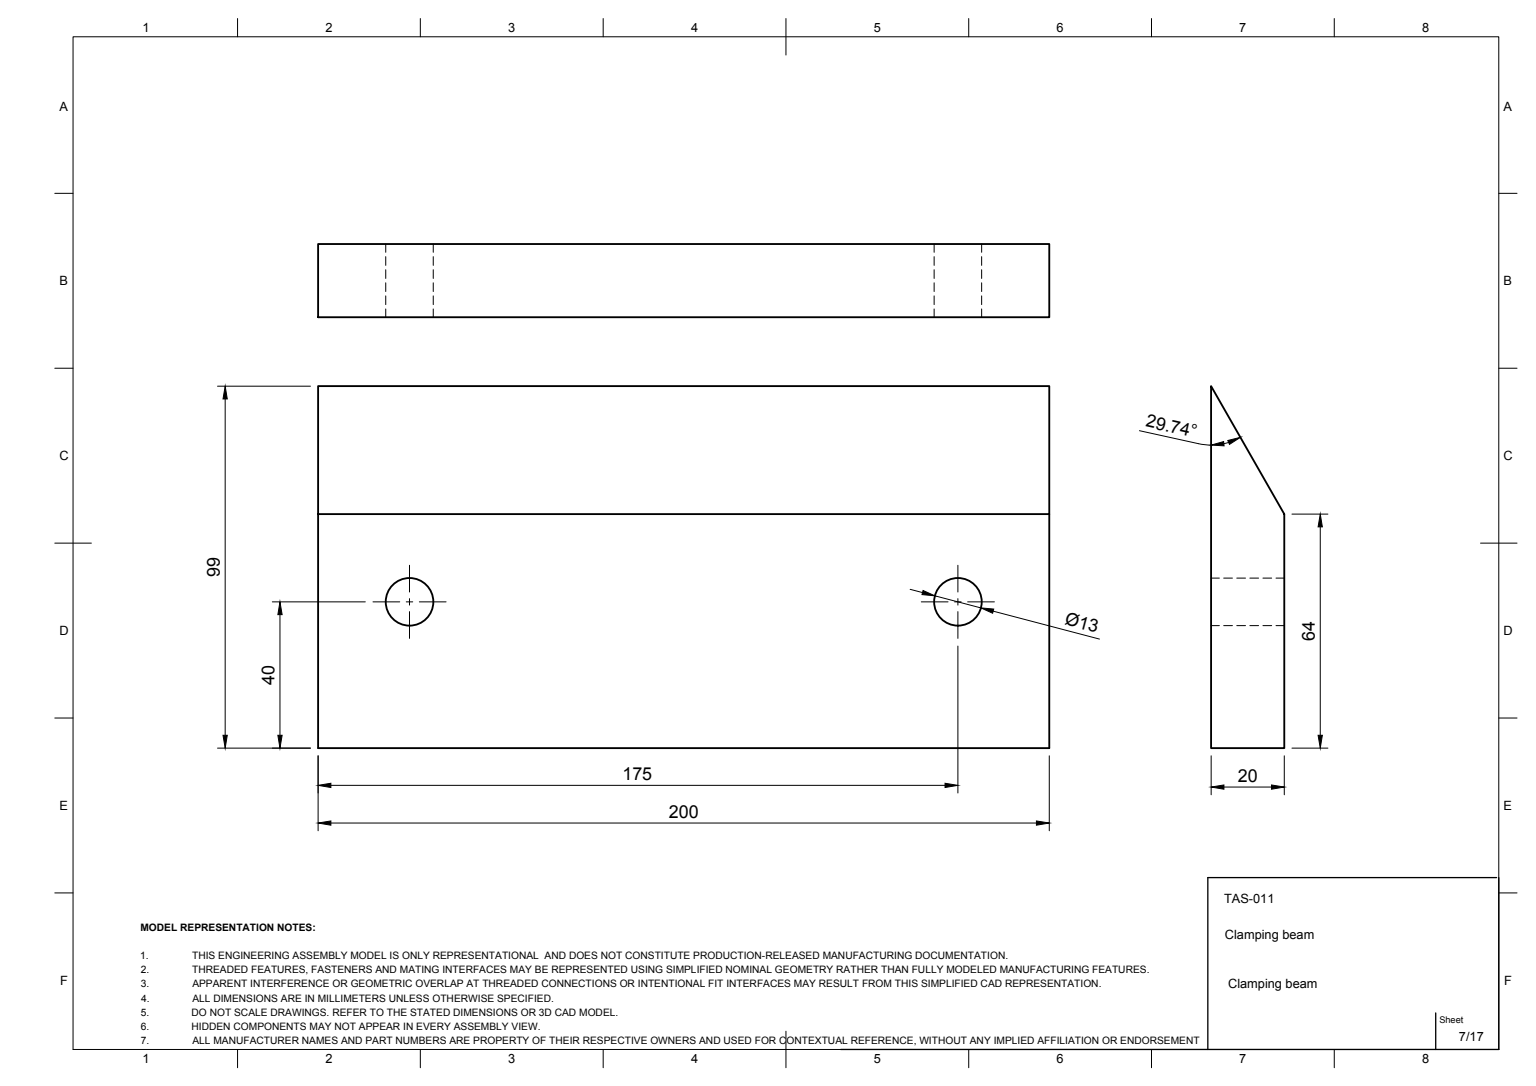
ISO-10303-21;
HEADER;
/* Generated by software containing ST-Developer
 * from STEP Tools, Inc. (www.steptools.com) 
 */

FILE_DESCRIPTION(
/* description */ (
'Independent manual bench leaf bending machine,200mm work width. Fabri
cated welded frame and folding leaf, repeated bushed and fully retaine
d hinge hardware, two handles with bonded grips, beveled clamping beam
 and modeledM12 clamp screws.2mm omitted-workpiece assembly reference 
gap, not a capacity claim. Native135deg hinge travel. Weld sizing, pro
duction fits, material condition, bending capacity, strength and life 
unassigned.'),
/* implementation_level */ '2;1');

FILE_NAME(
/* name */ 'Clamping beam.step',
/* time_stamp */ '2026-11-14T09:11:34-08:00',
/* author */ (''),
/* organization */ (''),
/* preprocessor_version */ 'ST-DEVELOPER v20.2',
/* originating_system */ 'Autodesk Translation Framework v15.17.0.0',
/* authorisation */ '');

FILE_SCHEMA (('AUTOMOTIVE_DESIGN { 1 0 10303 214 3 1 1 }'));
ENDSEC;

DATA;
#10=MECHANICAL_DESIGN_GEOMETRIC_PRESENTATION_REPRESENTATION('',(#448),#37701);
#412=SHAPE_REPRESENTATION_RELATIONSHIP('SRR','None',#37781,#430);
#430=ADVANCED_BREP_SHAPE_REPRESENTATION('',(#466),#37685);
#448=STYLED_ITEM('',(#37880),#466);
#466=MANIFOLD_SOLID_BREP('Body1',#4146);
#494=FACE_BOUND('',#852,.T.);
#495=FACE_BOUND('',#853,.T.);
#496=FACE_BOUND('',#856,.T.);
#497=FACE_BOUND('',#857,.T.);
#528=PLANE('',#4413);
#529=PLANE('',#4414);
#530=PLANE('',#4415);
#531=PLANE('',#4416);
#532=PLANE('',#4417);
#533=PLANE('',#4418);
#624=FACE_OUTER_BOUND('',#848,.T.);
#625=FACE_OUTER_BOUND('',#849,.T.);
#626=FACE_OUTER_BOUND('',#850,.T.);
#627=FACE_OUTER_BOUND('',#851,.T.);
#628=FACE_OUTER_BOUND('',#854,.T.);
#629=FACE_OUTER_BOUND('',#855,.T.);
#630=FACE_OUTER_BOUND('',#858,.T.);
#631=FACE_OUTER_BOUND('',#859,.T.);
#848=EDGE_LOOP('',(#2747,#2748,#2749,#2750));
#849=EDGE_LOOP('',(#2751,#2752,#2753,#2754));
#850=EDGE_LOOP('',(#2755,#2756,#2757,#2758));
#851=EDGE_LOOP('',(#2759,#2760,#2761,#2762));
#852=EDGE_LOOP('',(#2763));
#853=EDGE_LOOP('',(#2764));
#854=EDGE_LOOP('',(#2765,#2766,#2767,#2768));
#855=EDGE_LOOP('',(#2769,#2770,#2771,#2772));
#856=EDGE_LOOP('',(#2773));
#857=EDGE_LOOP('',(#2774));
#858=EDGE_LOOP('',(#2775,#2776,#2777,#2778));
#859=EDGE_LOOP('',(#2779,#2780,#2781,#2782));
#1094=LINE('',#5768,#1343);
#1095=LINE('',#5774,#1344);
#1096=LINE('',#5779,#1345);
#1097=LINE('',#5781,#1346);
#1098=LINE('',#5783,#1347);
#1099=LINE('',#5784,#1348);
#1100=LINE('',#5787,#1349);
#1101=LINE('',#5789,#1350);
#1102=LINE('',#5790,#1351);
#1103=LINE('',#5793,#1352);
#1104=LINE('',#5795,#1353);
#1105=LINE('',#5796,#1354);
#1106=LINE('',#5798,#1355);
#1107=LINE('',#5799,#1356);
#1343=VECTOR('',#4837,6.5);
#1344=VECTOR('',#4844,6.5);
#1345=VECTOR('',#4849,10.);
#1346=VECTOR('',#4850,10.);
#1347=VECTOR('',#4851,10.);
#1348=VECTOR('',#4852,10.);
#1349=VECTOR('',#4855,10.);
#1350=VECTOR('',#4856,10.);
#1351=VECTOR('',#4857,10.);
#1352=VECTOR('',#4860,10.);
#1353=VECTOR('',#4861,10.);
#1354=VECTOR('',#4862,10.);
#1355=VECTOR('',#4865,10.);
#1356=VECTOR('',#4866,10.);
#1578=CIRCLE('',#4408,6.5);
#1579=CIRCLE('',#4409,6.5);
#1580=CIRCLE('',#4411,6.5);
#1581=CIRCLE('',#4412,6.5);
#1673=VERTEX_POINT('',#5765);
#1674=VERTEX_POINT('',#5767);
#1675=VERTEX_POINT('',#5771);
#1676=VERTEX_POINT('',#5773);
#1677=VERTEX_POINT('',#5777);
#1678=VERTEX_POINT('',#5778);
#1679=VERTEX_POINT('',#5780);
#1680=VERTEX_POINT('',#5782);
#1681=VERTEX_POINT('',#5786);
#1682=VERTEX_POINT('',#5788);
#1683=VERTEX_POINT('',#5792);
#1684=VERTEX_POINT('',#5794);
#2107=EDGE_CURVE('',#1673,#1673,#1578,.T.);
#2108=EDGE_CURVE('',#1673,#1674,#1094,.T.);
#2109=EDGE_CURVE('',#1674,#1674,#1579,.T.);
#2110=EDGE_CURVE('',#1675,#1675,#1580,.T.);
#2111=EDGE_CURVE('',#1675,#1676,#1095,.T.);
#2112=EDGE_CURVE('',#1676,#1676,#1581,.T.);
#2113=EDGE_CURVE('',#1677,#1678,#1096,.T.);
#2114=EDGE_CURVE('',#1677,#1679,#1097,.T.);
#2115=EDGE_CURVE('',#1680,#1679,#1098,.T.);
#2116=EDGE_CURVE('',#1678,#1680,#1099,.T.);
#2117=EDGE_CURVE('',#1678,#1681,#1100,.T.);
#2118=EDGE_CURVE('',#1682,#1680,#1101,.T.);
#2119=EDGE_CURVE('',#1681,#1682,#1102,.T.);
#2120=EDGE_CURVE('',#1681,#1683,#1103,.T.);
#2121=EDGE_CURVE('',#1684,#1682,#1104,.T.);
#2122=EDGE_CURVE('',#1683,#1684,#1105,.T.);
#2123=EDGE_CURVE('',#1683,#1677,#1106,.T.);
#2124=EDGE_CURVE('',#1679,#1684,#1107,.T.);
#2747=ORIENTED_EDGE('',*,*,#2107,.F.);
#2748=ORIENTED_EDGE('',*,*,#2108,.T.);
#2749=ORIENTED_EDGE('',*,*,#2109,.F.);
#2750=ORIENTED_EDGE('',*,*,#2108,.F.);
#2751=ORIENTED_EDGE('',*,*,#2110,.F.);
#2752=ORIENTED_EDGE('',*,*,#2111,.T.);
#2753=ORIENTED_EDGE('',*,*,#2112,.F.);
#2754=ORIENTED_EDGE('',*,*,#2111,.F.);
#2755=ORIENTED_EDGE('',*,*,#2113,.F.);
#2756=ORIENTED_EDGE('',*,*,#2114,.T.);
#2757=ORIENTED_EDGE('',*,*,#2115,.F.);
#2758=ORIENTED_EDGE('',*,*,#2116,.F.);
#2759=ORIENTED_EDGE('',*,*,#2117,.F.);
#2760=ORIENTED_EDGE('',*,*,#2116,.T.);
#2761=ORIENTED_EDGE('',*,*,#2118,.F.);
#2762=ORIENTED_EDGE('',*,*,#2119,.F.);
#2763=ORIENTED_EDGE('',*,*,#2109,.T.);
#2764=ORIENTED_EDGE('',*,*,#2112,.T.);
#2765=ORIENTED_EDGE('',*,*,#2120,.F.);
#2766=ORIENTED_EDGE('',*,*,#2119,.T.);
#2767=ORIENTED_EDGE('',*,*,#2121,.F.);
#2768=ORIENTED_EDGE('',*,*,#2122,.F.);
#2769=ORIENTED_EDGE('',*,*,#2123,.F.);
#2770=ORIENTED_EDGE('',*,*,#2122,.T.);
#2771=ORIENTED_EDGE('',*,*,#2124,.F.);
#2772=ORIENTED_EDGE('',*,*,#2114,.F.);
#2773=ORIENTED_EDGE('',*,*,#2107,.T.);
#2774=ORIENTED_EDGE('',*,*,#2110,.T.);
#2775=ORIENTED_EDGE('',*,*,#2124,.T.);
#2776=ORIENTED_EDGE('',*,*,#2121,.T.);
#2777=ORIENTED_EDGE('',*,*,#2118,.T.);
#2778=ORIENTED_EDGE('',*,*,#2115,.T.);
#2779=ORIENTED_EDGE('',*,*,#2123,.T.);
#2780=ORIENTED_EDGE('',*,*,#2113,.T.);
#2781=ORIENTED_EDGE('',*,*,#2117,.T.);
#2782=ORIENTED_EDGE('',*,*,#2120,.T.);
#3821=CYLINDRICAL_SURFACE('',#4407,6.5);
#3822=CYLINDRICAL_SURFACE('',#4410,6.5);
#3954=ADVANCED_FACE('',(#624),#3821,.F.);
#3955=ADVANCED_FACE('',(#625),#3822,.F.);
#3956=ADVANCED_FACE('',(#626),#528,.T.);
#3957=ADVANCED_FACE('',(#627,#494,#495),#529,.T.);
#3958=ADVANCED_FACE('',(#628),#530,.T.);
#3959=ADVANCED_FACE('',(#629,#496,#497),#531,.T.);
#3960=ADVANCED_FACE('',(#630),#532,.T.);
#3961=ADVANCED_FACE('',(#631),#533,.F.);
#4146=CLOSED_SHELL('',(#3954,#3955,#3956,#3957,#3958,#3959,#3960,#3961));
#4406=AXIS2_PLACEMENT_3D('',#5763,#4831,#4832);
#4407=AXIS2_PLACEMENT_3D('',#5764,#4833,#4834);
#4408=AXIS2_PLACEMENT_3D('',#5766,#4835,#4836);
#4409=AXIS2_PLACEMENT_3D('',#5769,#4838,#4839);
#4410=AXIS2_PLACEMENT_3D('',#5770,#4840,#4841);
#4411=AXIS2_PLACEMENT_3D('',#5772,#4842,#4843);
#4412=AXIS2_PLACEMENT_3D('',#5775,#4845,#4846);
#4413=AXIS2_PLACEMENT_3D('',#5776,#4847,#4848);
#4414=AXIS2_PLACEMENT_3D('',#5785,#4853,#4854);
#4415=AXIS2_PLACEMENT_3D('',#5791,#4858,#4859);
#4416=AXIS2_PLACEMENT_3D('',#5797,#4863,#4864);
#4417=AXIS2_PLACEMENT_3D('',#5800,#4867,#4868);
#4418=AXIS2_PLACEMENT_3D('',#5801,#4869,#4870);
#4831=DIRECTION('axis',(0.,0.,1.));
#4832=DIRECTION('refdir',(1.,0.,0.));
#4833=DIRECTION('center_axis',(0.,0.,-1.));
#4834=DIRECTION('ref_axis',(1.,0.,0.));
#4835=DIRECTION('center_axis',(0.,0.,-1.));
#4836=DIRECTION('ref_axis',(1.,0.,0.));
#4837=DIRECTION('',(0.,0.,-1.));
#4838=DIRECTION('center_axis',(0.,0.,1.));
#4839=DIRECTION('ref_axis',(1.,0.,0.));
#4840=DIRECTION('center_axis',(0.,0.,-1.));
#4841=DIRECTION('ref_axis',(1.,0.,0.));
#4842=DIRECTION('center_axis',(0.,0.,-1.));
#4843=DIRECTION('ref_axis',(1.,0.,0.));
#4844=DIRECTION('',(0.,0.,-1.));
#4845=DIRECTION('center_axis',(0.,0.,1.));
#4846=DIRECTION('ref_axis',(1.,0.,0.));
#4847=DIRECTION('center_axis',(-1.,0.,0.));
#4848=DIRECTION('ref_axis',(0.,0.,1.));
#4849=DIRECTION('',(0.,0.,-1.));
#4850=DIRECTION('',(0.,1.,0.));
#4851=DIRECTION('',(0.,0.,1.));
#4852=DIRECTION('',(0.,1.,0.));
#4853=DIRECTION('center_axis',(0.,0.,-1.));
#4854=DIRECTION('ref_axis',(-1.,0.,0.));
#4855=DIRECTION('',(1.,0.,0.));
#4856=DIRECTION('',(-1.,0.,0.));
#4857=DIRECTION('',(0.,1.,0.));
#4858=DIRECTION('center_axis',(0.496138938356834,0.,0.868243142124459));
#4859=DIRECTION('ref_axis',(0.868243142124459,0.,-0.496138938356834));
#4860=DIRECTION('',(-0.868243142124459,0.,0.496138938356834));
#4861=DIRECTION('',(0.868243142124459,0.,-0.496138938356834));
#4862=DIRECTION('',(0.,1.,0.));
#4863=DIRECTION('center_axis',(0.,0.,1.));
#4864=DIRECTION('ref_axis',(1.,0.,0.));
#4865=DIRECTION('',(-1.,0.,0.));
#4866=DIRECTION('',(1.,0.,0.));
#4867=DIRECTION('center_axis',(0.,1.,0.));
#4868=DIRECTION('ref_axis',(0.,0.,1.));
#4869=DIRECTION('center_axis',(0.,1.,0.));
#4870=DIRECTION('ref_axis',(1.,0.,0.));
#5763=CARTESIAN_POINT('',(0.,0.,0.));
#5764=CARTESIAN_POINT('Origin',(-60.,25.,52.));
#5765=CARTESIAN_POINT('',(-66.5,25.,62.));
#5766=CARTESIAN_POINT('Origin',(-60.,25.,62.));
#5767=CARTESIAN_POINT('',(-66.5,25.,42.));
#5768=CARTESIAN_POINT('',(-66.5,25.,52.));
#5769=CARTESIAN_POINT('Origin',(-60.,25.,42.));
#5770=CARTESIAN_POINT('Origin',(-60.,175.,52.));
#5771=CARTESIAN_POINT('',(-66.5,175.,62.));
#5772=CARTESIAN_POINT('Origin',(-60.,175.,62.));
#5773=CARTESIAN_POINT('',(-66.5,175.,42.));
#5774=CARTESIAN_POINT('',(-66.5,175.,52.));
#5775=CARTESIAN_POINT('Origin',(-60.,175.,42.));
#5776=CARTESIAN_POINT('Origin',(-100.,0.,42.));
#5777=CARTESIAN_POINT('',(-100.,0.,62.));
#5778=CARTESIAN_POINT('',(-100.,0.,42.));
#5779=CARTESIAN_POINT('',(-100.,0.,62.));
#5780=CARTESIAN_POINT('',(-100.,200.,62.));
#5781=CARTESIAN_POINT('',(-100.,0.,62.));
#5782=CARTESIAN_POINT('',(-100.,200.,42.));
#5783=CARTESIAN_POINT('',(-100.,200.,62.));
#5784=CARTESIAN_POINT('',(-100.,0.,42.));
#5785=CARTESIAN_POINT('Origin',(-0.999999999999996,0.,42.));
#5786=CARTESIAN_POINT('',(-1.,0.,42.));
#5787=CARTESIAN_POINT('',(-100.,0.,42.));
#5788=CARTESIAN_POINT('',(-1.,200.,42.));
#5789=CARTESIAN_POINT('',(-100.,200.,42.));
#5790=CARTESIAN_POINT('',(-1.,0.,42.));
#5791=CARTESIAN_POINT('Origin',(-36.,0.,62.));
#5792=CARTESIAN_POINT('',(-36.,0.,62.));
#5793=CARTESIAN_POINT('',(-1.,0.,42.));
#5794=CARTESIAN_POINT('',(-36.,200.,62.));
#5795=CARTESIAN_POINT('',(-1.,200.,42.));
#5796=CARTESIAN_POINT('',(-36.,0.,62.));
#5797=CARTESIAN_POINT('Origin',(-100.,0.,62.));
#5798=CARTESIAN_POINT('',(-36.,0.,62.));
#5799=CARTESIAN_POINT('',(-36.,200.,62.));
#5800=CARTESIAN_POINT('Origin',(-50.5,200.,52.));
#5801=CARTESIAN_POINT('Origin',(-50.5,0.,52.));
#37665=UNCERTAINTY_MEASURE_WITH_UNIT(LENGTH_MEASURE(0.01),#37702,
'DISTANCE_ACCURACY_VALUE',
'Maximum model space distance between geometric entities at asserted c
onnectivities');
#37681=UNCERTAINTY_MEASURE_WITH_UNIT(LENGTH_MEASURE(0.01),#37702,
'DISTANCE_ACCURACY_VALUE',
'Maximum model space distance between geometric entities at asserted c
onnectivities');
#37685=(
GEOMETRIC_REPRESENTATION_CONTEXT(3)
GLOBAL_UNCERTAINTY_ASSIGNED_CONTEXT((#37665))
GLOBAL_UNIT_ASSIGNED_CONTEXT((#37702,#37704,#37705))
REPRESENTATION_CONTEXT('','3D')
);
#37701=(
GEOMETRIC_REPRESENTATION_CONTEXT(3)
GLOBAL_UNCERTAINTY_ASSIGNED_CONTEXT((#37681))
GLOBAL_UNIT_ASSIGNED_CONTEXT((#37702,#37704,#37705))
REPRESENTATION_CONTEXT('','3D')
);
#37702=(
LENGTH_UNIT()
NAMED_UNIT(*)
SI_UNIT(.MILLI.,.METRE.)
);
#37704=(
NAMED_UNIT(*)
PLANE_ANGLE_UNIT()
SI_UNIT($,.RADIAN.)
);
#37705=(
NAMED_UNIT(*)
SI_UNIT($,.STERADIAN.)
SOLID_ANGLE_UNIT()
);
#37709=SHAPE_DEFINITION_REPRESENTATION(#37728,#37781);
#37728=PRODUCT_DEFINITION_SHAPE('',$,#37801);
#37781=SHAPE_REPRESENTATION('',(#4406),#37685);
#37797=PRODUCT_DEFINITION_CONTEXT('part definition',#37856,'design');
#37801=PRODUCT_DEFINITION('Clamping beam','Clamping beam',#37820,#37797);
#37820=PRODUCT_DEFINITION_FORMATION('',$,#37861);
#37856=APPLICATION_CONTEXT(
'Core Data for Automotive Mechanical Design Process');
#37857=PRODUCT_CONTEXT('part definition',#37856,'mechanical');
#37861=PRODUCT('Clamping beam','Clamping beam',$,(#37857));
#37880=PRESENTATION_STYLE_ASSIGNMENT((#37888));
#37888=SURFACE_STYLE_USAGE(.BOTH.,#37896);
#37896=SURFACE_SIDE_STYLE('',(#37904));
#37904=SURFACE_STYLE_FILL_AREA(#37912);
#37912=FILL_AREA_STYLE('Opaque(185,192,202)',(#37920));
#37920=FILL_AREA_STYLE_COLOUR('Opaque(185,192,202)',#37928);
#37928=COLOUR_RGB('Opaque(185,192,202)',0.725490196078431,0.752941176470588,
0.792156862745098);
ENDSEC;
END-ISO-10303-21;
